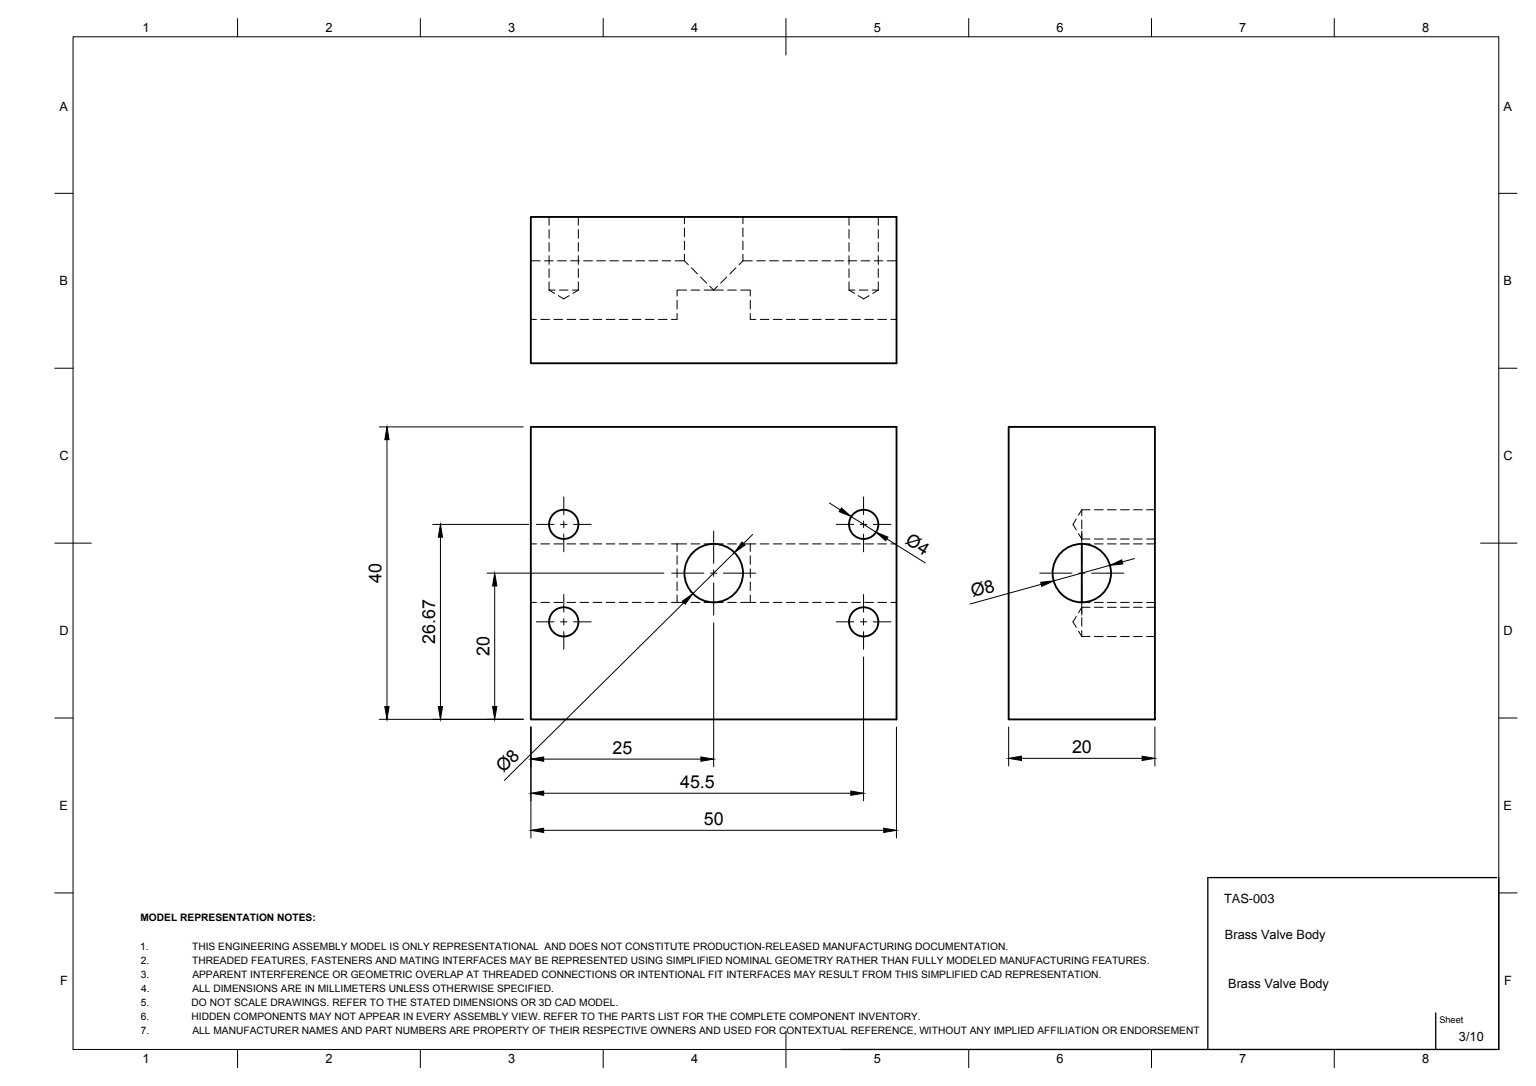
ISO-10303-21;
HEADER;
/* Generated by software containing ST-Developer
 * from STEP Tools, Inc. (www.steptools.com) 
 */

FILE_DESCRIPTION(
/* description */ ('STEP AP214'),
/* implementation_level */ '2;1');

FILE_NAME(
/* name */ 'Brass Valve Body.step',
/* time_stamp */ '2026-11-04T19:43:37-08:00',
/* author */ (''),
/* organization */ (''),
/* preprocessor_version */ 'ST-DEVELOPER v20.2',
/* originating_system */ 'Autodesk Translation Framework v15.17.0.0',
/* authorisation */ '');

FILE_SCHEMA (('AUTOMOTIVE_DESIGN { 1 0 10303 214 3 1 1 }'));
ENDSEC;

DATA;
#10=MECHANICAL_DESIGN_GEOMETRIC_PRESENTATION_REPRESENTATION('',(#115),#7627);
#97=SHAPE_REPRESENTATION_RELATIONSHIP('SRR','None',#7665,#106);
#106=ADVANCED_BREP_SHAPE_REPRESENTATION('',(#136),#7618);
#115=STYLED_ITEM('',(#7719),#136);
#136=MANIFOLD_SOLID_BREP('Body1',#2413);
#157=FACE_BOUND('',#474,.T.);
#158=FACE_BOUND('',#476,.T.);
#159=FACE_BOUND('',#479,.T.);
#160=FACE_BOUND('',#480,.T.);
#161=FACE_BOUND('',#481,.T.);
#162=FACE_BOUND('',#482,.T.);
#163=FACE_BOUND('',#483,.T.);
#191=PLANE('',#2563);
#192=PLANE('',#2564);
#193=PLANE('',#2565);
#194=PLANE('',#2566);
#195=PLANE('',#2567);
#196=PLANE('',#2568);
#197=PLANE('',#2569);
#198=PLANE('',#2570);
#199=PLANE('',#2571);
#252=ELLIPSE('',#2553,5.6568542494923,3.99999999999995);
#253=ELLIPSE('',#2554,5.65685424949242,4.00000000000003);
#254=ELLIPSE('',#2556,5.65685424949242,4.00000000000003);
#255=CYLINDRICAL_SURFACE('',#2538,2.);
#256=CYLINDRICAL_SURFACE('',#2542,2.);
#257=CYLINDRICAL_SURFACE('',#2546,2.);
#258=CYLINDRICAL_SURFACE('',#2550,2.);
#259=CYLINDRICAL_SURFACE('',#2552,4.);
#260=CYLINDRICAL_SURFACE('',#2557,4.);
#261=CYLINDRICAL_SURFACE('',#2560,4.);
#308=FACE_OUTER_BOUND('',#462,.T.);
#309=FACE_OUTER_BOUND('',#463,.T.);
#310=FACE_OUTER_BOUND('',#464,.T.);
#311=FACE_OUTER_BOUND('',#465,.T.);
#312=FACE_OUTER_BOUND('',#466,.T.);
#313=FACE_OUTER_BOUND('',#467,.T.);
#314=FACE_OUTER_BOUND('',#468,.T.);
#315=FACE_OUTER_BOUND('',#469,.T.);
#316=FACE_OUTER_BOUND('',#470,.T.);
#317=FACE_OUTER_BOUND('',#471,.T.);
#318=FACE_OUTER_BOUND('',#472,.T.);
#319=FACE_OUTER_BOUND('',#473,.T.);
#320=FACE_OUTER_BOUND('',#475,.T.);
#321=FACE_OUTER_BOUND('',#477,.T.);
#322=FACE_OUTER_BOUND('',#478,.T.);
#323=FACE_OUTER_BOUND('',#484,.T.);
#324=FACE_OUTER_BOUND('',#485,.T.);
#325=FACE_OUTER_BOUND('',#486,.T.);
#326=FACE_OUTER_BOUND('',#487,.T.);
#327=FACE_OUTER_BOUND('',#488,.T.);
#462=EDGE_LOOP('',(#1621,#1622,#1623));
#463=EDGE_LOOP('',(#1624,#1625,#1626,#1627));
#464=EDGE_LOOP('',(#1628,#1629,#1630));
#465=EDGE_LOOP('',(#1631,#1632,#1633,#1634));
#466=EDGE_LOOP('',(#1635,#1636,#1637));
#467=EDGE_LOOP('',(#1638,#1639,#1640,#1641));
#468=EDGE_LOOP('',(#1642,#1643,#1644));
#469=EDGE_LOOP('',(#1645,#1646,#1647,#1648));
#470=EDGE_LOOP('',(#1649,#1650,#1651,#1652,#1653,#1654));
#471=EDGE_LOOP('',(#1655,#1656,#1657,#1658,#1659,#1660,#1661,#1662));
#472=EDGE_LOOP('',(#1663,#1664,#1665,#1666,#1667,#1668,#1669));
#473=EDGE_LOOP('',(#1670,#1671,#1672,#1673));
#474=EDGE_LOOP('',(#1674));
#475=EDGE_LOOP('',(#1675,#1676,#1677,#1678));
#476=EDGE_LOOP('',(#1679));
#477=EDGE_LOOP('',(#1680,#1681,#1682,#1683));
#478=EDGE_LOOP('',(#1684,#1685,#1686,#1687));
#479=EDGE_LOOP('',(#1688));
#480=EDGE_LOOP('',(#1689));
#481=EDGE_LOOP('',(#1690));
#482=EDGE_LOOP('',(#1691));
#483=EDGE_LOOP('',(#1692));
#484=EDGE_LOOP('',(#1693,#1694,#1695,#1696));
#485=EDGE_LOOP('',(#1697,#1698,#1699,#1700));
#486=EDGE_LOOP('',(#1701,#1702));
#487=EDGE_LOOP('',(#1703,#1704));
#488=EDGE_LOOP('',(#1705,#1706,#1707,#1708,#1709,#1710));
#650=CIRCLE('',#2537,2.);
#651=CIRCLE('',#2539,2.);
#652=CIRCLE('',#2541,2.);
#653=CIRCLE('',#2543,2.);
#654=CIRCLE('',#2545,2.);
#655=CIRCLE('',#2547,2.);
#656=CIRCLE('',#2549,2.);
#657=CIRCLE('',#2551,2.);
#658=CIRCLE('',#2555,4.);
#659=CIRCLE('',#2558,4.);
#660=CIRCLE('',#2559,4.);
#661=CIRCLE('',#2561,4.);
#662=CIRCLE('',#2562,4.);
#803=LINE('',#3685,#959);
#804=LINE('',#3689,#960);
#805=LINE('',#3694,#961);
#806=LINE('',#3698,#962);
#807=LINE('',#3703,#963);
#808=LINE('',#3707,#964);
#809=LINE('',#3712,#965);
#810=LINE('',#3716,#966);
#811=LINE('',#3725,#967);
#812=LINE('',#3733,#968);
#813=LINE('',#3735,#969);
#814=LINE('',#3736,#970);
#815=LINE('',#3741,#971);
#816=LINE('',#3744,#972);
#817=LINE('',#3745,#973);
#818=LINE('',#3749,#974);
#819=LINE('',#3751,#975);
#820=LINE('',#3753,#976);
#821=LINE('',#3754,#977);
#822=LINE('',#3758,#978);
#823=LINE('',#3760,#979);
#824=LINE('',#3762,#980);
#825=LINE('',#3763,#981);
#826=LINE('',#3765,#982);
#827=LINE('',#3766,#983);
#828=LINE('',#3768,#984);
#829=LINE('',#3770,#985);
#830=LINE('',#3773,#986);
#831=LINE('',#3775,#987);
#959=VECTOR('',#2870,2.);
#960=VECTOR('',#2875,2.);
#961=VECTOR('',#2880,2.);
#962=VECTOR('',#2885,2.);
#963=VECTOR('',#2890,2.);
#964=VECTOR('',#2895,2.);
#965=VECTOR('',#2900,2.);
#966=VECTOR('',#2905,2.);
#967=VECTOR('',#2914,4.);
#968=VECTOR('',#2923,4.);
#969=VECTOR('',#2926,1000.);
#970=VECTOR('',#2927,1000.);
#971=VECTOR('',#2932,4.);
#972=VECTOR('',#2935,1000.);
#973=VECTOR('',#2936,1000.);
#974=VECTOR('',#2939,1000.);
#975=VECTOR('',#2940,1000.);
#976=VECTOR('',#2941,1000.);
#977=VECTOR('',#2942,1000.);
#978=VECTOR('',#2945,1000.);
#979=VECTOR('',#2946,1000.);
#980=VECTOR('',#2947,1000.);
#981=VECTOR('',#2948,1000.);
#982=VECTOR('',#2951,1000.);
#983=VECTOR('',#2952,1000.);
#984=VECTOR('',#2955,1000.);
#985=VECTOR('',#2958,1000.);
#986=VECTOR('',#2963,1000.);
#987=VECTOR('',#2966,1000.);
#1115=VERTEX_POINT('',#3683);
#1116=VERTEX_POINT('',#3684);
#1117=VERTEX_POINT('',#3688);
#1118=VERTEX_POINT('',#3692);
#1119=VERTEX_POINT('',#3693);
#1120=VERTEX_POINT('',#3697);
#1121=VERTEX_POINT('',#3701);
#1122=VERTEX_POINT('',#3702);
#1123=VERTEX_POINT('',#3706);
#1124=VERTEX_POINT('',#3710);
#1125=VERTEX_POINT('',#3711);
#1126=VERTEX_POINT('',#3715);
#1127=VERTEX_POINT('',#3719);
#1128=VERTEX_POINT('',#3720);
#1129=VERTEX_POINT('',#3722);
#1130=VERTEX_POINT('',#3724);
#1131=VERTEX_POINT('',#3729);
#1132=VERTEX_POINT('',#3730);
#1133=VERTEX_POINT('',#3732);
#1134=VERTEX_POINT('',#3738);
#1135=VERTEX_POINT('',#3740);
#1136=VERTEX_POINT('',#3742);
#1137=VERTEX_POINT('',#3747);
#1138=VERTEX_POINT('',#3748);
#1139=VERTEX_POINT('',#3750);
#1140=VERTEX_POINT('',#3752);
#1141=VERTEX_POINT('',#3756);
#1142=VERTEX_POINT('',#3757);
#1143=VERTEX_POINT('',#3759);
#1144=VERTEX_POINT('',#3761);
#1305=EDGE_CURVE('',#1115,#1116,#803,.T.);
#1306=EDGE_CURVE('',#1116,#1116,#650,.T.);
#1307=EDGE_CURVE('',#1116,#1117,#804,.T.);
#1308=EDGE_CURVE('',#1117,#1117,#651,.T.);
#1309=EDGE_CURVE('',#1118,#1119,#805,.T.);
#1310=EDGE_CURVE('',#1119,#1119,#652,.T.);
#1311=EDGE_CURVE('',#1119,#1120,#806,.T.);
#1312=EDGE_CURVE('',#1120,#1120,#653,.T.);
#1313=EDGE_CURVE('',#1121,#1122,#807,.T.);
#1314=EDGE_CURVE('',#1122,#1122,#654,.T.);
#1315=EDGE_CURVE('',#1122,#1123,#808,.T.);
#1316=EDGE_CURVE('',#1123,#1123,#655,.T.);
#1317=EDGE_CURVE('',#1124,#1125,#809,.T.);
#1318=EDGE_CURVE('',#1125,#1125,#656,.T.);
#1319=EDGE_CURVE('',#1125,#1126,#810,.T.);
#1320=EDGE_CURVE('',#1126,#1126,#657,.T.);
#1321=EDGE_CURVE('',#1127,#1128,#252,.T.);
#1322=EDGE_CURVE('',#1129,#1127,#253,.T.);
#1323=EDGE_CURVE('',#1129,#1130,#811,.T.);
#1324=EDGE_CURVE('',#1130,#1130,#658,.T.);
#1325=EDGE_CURVE('',#1128,#1129,#254,.T.);
#1326=EDGE_CURVE('',#1131,#1132,#659,.T.);
#1327=EDGE_CURVE('',#1131,#1133,#812,.T.);
#1328=EDGE_CURVE('',#1133,#1133,#660,.T.);
#1329=EDGE_CURVE('',#1128,#1131,#813,.T.);
#1330=EDGE_CURVE('',#1132,#1127,#814,.T.);
#1331=EDGE_CURVE('',#1134,#1134,#661,.T.);
#1332=EDGE_CURVE('',#1134,#1135,#815,.T.);
#1333=EDGE_CURVE('',#1136,#1135,#662,.T.);
#1334=EDGE_CURVE('',#1127,#1136,#816,.T.);
#1335=EDGE_CURVE('',#1135,#1128,#817,.T.);
#1336=EDGE_CURVE('',#1137,#1138,#818,.T.);
#1337=EDGE_CURVE('',#1138,#1139,#819,.T.);
#1338=EDGE_CURVE('',#1139,#1140,#820,.T.);
#1339=EDGE_CURVE('',#1140,#1137,#821,.T.);
#1340=EDGE_CURVE('',#1141,#1142,#822,.T.);
#1341=EDGE_CURVE('',#1143,#1141,#823,.T.);
#1342=EDGE_CURVE('',#1144,#1143,#824,.T.);
#1343=EDGE_CURVE('',#1142,#1144,#825,.T.);
#1344=EDGE_CURVE('',#1138,#1142,#826,.T.);
#1345=EDGE_CURVE('',#1137,#1141,#827,.T.);
#1346=EDGE_CURVE('',#1139,#1144,#828,.T.);
#1347=EDGE_CURVE('',#1140,#1143,#829,.T.);
#1348=EDGE_CURVE('',#1132,#1131,#830,.T.);
#1349=EDGE_CURVE('',#1135,#1136,#831,.T.);
#1621=ORIENTED_EDGE('',*,*,#1305,.T.);
#1622=ORIENTED_EDGE('',*,*,#1306,.T.);
#1623=ORIENTED_EDGE('',*,*,#1305,.F.);
#1624=ORIENTED_EDGE('',*,*,#1306,.F.);
#1625=ORIENTED_EDGE('',*,*,#1307,.T.);
#1626=ORIENTED_EDGE('',*,*,#1308,.T.);
#1627=ORIENTED_EDGE('',*,*,#1307,.F.);
#1628=ORIENTED_EDGE('',*,*,#1309,.T.);
#1629=ORIENTED_EDGE('',*,*,#1310,.T.);
#1630=ORIENTED_EDGE('',*,*,#1309,.F.);
#1631=ORIENTED_EDGE('',*,*,#1310,.F.);
#1632=ORIENTED_EDGE('',*,*,#1311,.T.);
#1633=ORIENTED_EDGE('',*,*,#1312,.T.);
#1634=ORIENTED_EDGE('',*,*,#1311,.F.);
#1635=ORIENTED_EDGE('',*,*,#1313,.T.);
#1636=ORIENTED_EDGE('',*,*,#1314,.T.);
#1637=ORIENTED_EDGE('',*,*,#1313,.F.);
#1638=ORIENTED_EDGE('',*,*,#1314,.F.);
#1639=ORIENTED_EDGE('',*,*,#1315,.T.);
#1640=ORIENTED_EDGE('',*,*,#1316,.T.);
#1641=ORIENTED_EDGE('',*,*,#1315,.F.);
#1642=ORIENTED_EDGE('',*,*,#1317,.T.);
#1643=ORIENTED_EDGE('',*,*,#1318,.T.);
#1644=ORIENTED_EDGE('',*,*,#1317,.F.);
#1645=ORIENTED_EDGE('',*,*,#1318,.F.);
#1646=ORIENTED_EDGE('',*,*,#1319,.T.);
#1647=ORIENTED_EDGE('',*,*,#1320,.T.);
#1648=ORIENTED_EDGE('',*,*,#1319,.F.);
#1649=ORIENTED_EDGE('',*,*,#1321,.F.);
#1650=ORIENTED_EDGE('',*,*,#1322,.F.);
#1651=ORIENTED_EDGE('',*,*,#1323,.T.);
#1652=ORIENTED_EDGE('',*,*,#1324,.T.);
#1653=ORIENTED_EDGE('',*,*,#1323,.F.);
#1654=ORIENTED_EDGE('',*,*,#1325,.F.);
#1655=ORIENTED_EDGE('',*,*,#1326,.F.);
#1656=ORIENTED_EDGE('',*,*,#1327,.T.);
#1657=ORIENTED_EDGE('',*,*,#1328,.F.);
#1658=ORIENTED_EDGE('',*,*,#1327,.F.);
#1659=ORIENTED_EDGE('',*,*,#1329,.F.);
#1660=ORIENTED_EDGE('',*,*,#1325,.T.);
#1661=ORIENTED_EDGE('',*,*,#1322,.T.);
#1662=ORIENTED_EDGE('',*,*,#1330,.F.);
#1663=ORIENTED_EDGE('',*,*,#1331,.T.);
#1664=ORIENTED_EDGE('',*,*,#1332,.T.);
#1665=ORIENTED_EDGE('',*,*,#1333,.F.);
#1666=ORIENTED_EDGE('',*,*,#1334,.F.);
#1667=ORIENTED_EDGE('',*,*,#1321,.T.);
#1668=ORIENTED_EDGE('',*,*,#1335,.F.);
#1669=ORIENTED_EDGE('',*,*,#1332,.F.);
#1670=ORIENTED_EDGE('',*,*,#1336,.T.);
#1671=ORIENTED_EDGE('',*,*,#1337,.T.);
#1672=ORIENTED_EDGE('',*,*,#1338,.T.);
#1673=ORIENTED_EDGE('',*,*,#1339,.T.);
#1674=ORIENTED_EDGE('',*,*,#1331,.F.);
#1675=ORIENTED_EDGE('',*,*,#1340,.F.);
#1676=ORIENTED_EDGE('',*,*,#1341,.F.);
#1677=ORIENTED_EDGE('',*,*,#1342,.F.);
#1678=ORIENTED_EDGE('',*,*,#1343,.F.);
#1679=ORIENTED_EDGE('',*,*,#1328,.T.);
#1680=ORIENTED_EDGE('',*,*,#1340,.T.);
#1681=ORIENTED_EDGE('',*,*,#1344,.F.);
#1682=ORIENTED_EDGE('',*,*,#1336,.F.);
#1683=ORIENTED_EDGE('',*,*,#1345,.T.);
#1684=ORIENTED_EDGE('',*,*,#1343,.T.);
#1685=ORIENTED_EDGE('',*,*,#1346,.F.);
#1686=ORIENTED_EDGE('',*,*,#1337,.F.);
#1687=ORIENTED_EDGE('',*,*,#1344,.T.);
#1688=ORIENTED_EDGE('',*,*,#1308,.F.);
#1689=ORIENTED_EDGE('',*,*,#1312,.F.);
#1690=ORIENTED_EDGE('',*,*,#1316,.F.);
#1691=ORIENTED_EDGE('',*,*,#1320,.F.);
#1692=ORIENTED_EDGE('',*,*,#1324,.F.);
#1693=ORIENTED_EDGE('',*,*,#1342,.T.);
#1694=ORIENTED_EDGE('',*,*,#1347,.F.);
#1695=ORIENTED_EDGE('',*,*,#1338,.F.);
#1696=ORIENTED_EDGE('',*,*,#1346,.T.);
#1697=ORIENTED_EDGE('',*,*,#1341,.T.);
#1698=ORIENTED_EDGE('',*,*,#1345,.F.);
#1699=ORIENTED_EDGE('',*,*,#1339,.F.);
#1700=ORIENTED_EDGE('',*,*,#1347,.T.);
#1701=ORIENTED_EDGE('',*,*,#1348,.T.);
#1702=ORIENTED_EDGE('',*,*,#1326,.T.);
#1703=ORIENTED_EDGE('',*,*,#1349,.T.);
#1704=ORIENTED_EDGE('',*,*,#1333,.T.);
#1705=ORIENTED_EDGE('',*,*,#1349,.F.);
#1706=ORIENTED_EDGE('',*,*,#1335,.T.);
#1707=ORIENTED_EDGE('',*,*,#1329,.T.);
#1708=ORIENTED_EDGE('',*,*,#1348,.F.);
#1709=ORIENTED_EDGE('',*,*,#1330,.T.);
#1710=ORIENTED_EDGE('',*,*,#1334,.T.);
#2253=CONICAL_SURFACE('',#2536,2.,1.02974426);
#2254=CONICAL_SURFACE('',#2540,2.,1.02974426);
#2255=CONICAL_SURFACE('',#2544,2.,1.02974426);
#2256=CONICAL_SURFACE('',#2548,2.,1.02974426);
#2259=ADVANCED_FACE('',(#308),#2253,.F.);
#2260=ADVANCED_FACE('',(#309),#255,.F.);
#2261=ADVANCED_FACE('',(#310),#2254,.F.);
#2262=ADVANCED_FACE('',(#311),#256,.F.);
#2263=ADVANCED_FACE('',(#312),#2255,.F.);
#2264=ADVANCED_FACE('',(#313),#257,.F.);
#2265=ADVANCED_FACE('',(#314),#2256,.F.);
#2266=ADVANCED_FACE('',(#315),#258,.F.);
#2267=ADVANCED_FACE('',(#316),#259,.F.);
#2268=ADVANCED_FACE('',(#317),#260,.F.);
#2269=ADVANCED_FACE('',(#318),#261,.F.);
#2270=ADVANCED_FACE('',(#319,#157),#191,.F.);
#2271=ADVANCED_FACE('',(#320,#158),#192,.T.);
#2272=ADVANCED_FACE('',(#321),#193,.F.);
#2273=ADVANCED_FACE('',(#322,#159,#160,#161,#162,#163),#194,.F.);
#2274=ADVANCED_FACE('',(#323),#195,.F.);
#2275=ADVANCED_FACE('',(#324),#196,.F.);
#2276=ADVANCED_FACE('',(#325),#197,.T.);
#2277=ADVANCED_FACE('',(#326),#198,.T.);
#2278=ADVANCED_FACE('',(#327),#199,.T.);
#2413=CLOSED_SHELL('',(#2259,#2260,#2261,#2262,#2263,#2264,#2265,#2266,
#2267,#2268,#2269,#2270,#2271,#2272,#2273,#2274,#2275,#2276,#2277,#2278));
#2535=AXIS2_PLACEMENT_3D('',#3681,#2866,#2867);
#2536=AXIS2_PLACEMENT_3D('',#3682,#2868,#2869);
#2537=AXIS2_PLACEMENT_3D('',#3686,#2871,#2872);
#2538=AXIS2_PLACEMENT_3D('',#3687,#2873,#2874);
#2539=AXIS2_PLACEMENT_3D('',#3690,#2876,#2877);
#2540=AXIS2_PLACEMENT_3D('',#3691,#2878,#2879);
#2541=AXIS2_PLACEMENT_3D('',#3695,#2881,#2882);
#2542=AXIS2_PLACEMENT_3D('',#3696,#2883,#2884);
#2543=AXIS2_PLACEMENT_3D('',#3699,#2886,#2887);
#2544=AXIS2_PLACEMENT_3D('',#3700,#2888,#2889);
#2545=AXIS2_PLACEMENT_3D('',#3704,#2891,#2892);
#2546=AXIS2_PLACEMENT_3D('',#3705,#2893,#2894);
#2547=AXIS2_PLACEMENT_3D('',#3708,#2896,#2897);
#2548=AXIS2_PLACEMENT_3D('',#3709,#2898,#2899);
#2549=AXIS2_PLACEMENT_3D('',#3713,#2901,#2902);
#2550=AXIS2_PLACEMENT_3D('',#3714,#2903,#2904);
#2551=AXIS2_PLACEMENT_3D('',#3717,#2906,#2907);
#2552=AXIS2_PLACEMENT_3D('',#3718,#2908,#2909);
#2553=AXIS2_PLACEMENT_3D('',#3721,#2910,#2911);
#2554=AXIS2_PLACEMENT_3D('',#3723,#2912,#2913);
#2555=AXIS2_PLACEMENT_3D('',#3726,#2915,#2916);
#2556=AXIS2_PLACEMENT_3D('',#3727,#2917,#2918);
#2557=AXIS2_PLACEMENT_3D('',#3728,#2919,#2920);
#2558=AXIS2_PLACEMENT_3D('',#3731,#2921,#2922);
#2559=AXIS2_PLACEMENT_3D('',#3734,#2924,#2925);
#2560=AXIS2_PLACEMENT_3D('',#3737,#2928,#2929);
#2561=AXIS2_PLACEMENT_3D('',#3739,#2930,#2931);
#2562=AXIS2_PLACEMENT_3D('',#3743,#2933,#2934);
#2563=AXIS2_PLACEMENT_3D('',#3746,#2937,#2938);
#2564=AXIS2_PLACEMENT_3D('',#3755,#2943,#2944);
#2565=AXIS2_PLACEMENT_3D('',#3764,#2949,#2950);
#2566=AXIS2_PLACEMENT_3D('',#3767,#2953,#2954);
#2567=AXIS2_PLACEMENT_3D('',#3769,#2956,#2957);
#2568=AXIS2_PLACEMENT_3D('',#3771,#2959,#2960);
#2569=AXIS2_PLACEMENT_3D('',#3772,#2961,#2962);
#2570=AXIS2_PLACEMENT_3D('',#3774,#2964,#2965);
#2571=AXIS2_PLACEMENT_3D('',#3776,#2967,#2968);
#2866=DIRECTION('axis',(0.,0.,1.));
#2867=DIRECTION('refdir',(1.,0.,0.));
#2868=DIRECTION('center_axis',(0.,1.,0.));
#2869=DIRECTION('ref_axis',(0.,0.,1.));
#2870=DIRECTION('',(-1.04972719197331E-16,0.515038073775726,-0.857167301383686));
#2871=DIRECTION('center_axis',(0.,1.,0.));
#2872=DIRECTION('ref_axis',(0.,0.,1.));
#2873=DIRECTION('center_axis',(0.,1.,0.));
#2874=DIRECTION('ref_axis',(0.,0.,1.));
#2875=DIRECTION('',(0.,1.,0.));
#2876=DIRECTION('center_axis',(0.,1.,0.));
#2877=DIRECTION('ref_axis',(0.,0.,1.));
#2878=DIRECTION('center_axis',(0.,1.,0.));
#2879=DIRECTION('ref_axis',(0.,0.,1.));
#2880=DIRECTION('',(-1.04972719197331E-16,0.515038073775726,-0.857167301383686));
#2881=DIRECTION('center_axis',(0.,1.,0.));
#2882=DIRECTION('ref_axis',(0.,0.,1.));
#2883=DIRECTION('center_axis',(0.,1.,0.));
#2884=DIRECTION('ref_axis',(0.,0.,1.));
#2885=DIRECTION('',(0.,1.,0.));
#2886=DIRECTION('center_axis',(0.,1.,0.));
#2887=DIRECTION('ref_axis',(0.,0.,1.));
#2888=DIRECTION('center_axis',(0.,1.,0.));
#2889=DIRECTION('ref_axis',(0.,0.,1.));
#2890=DIRECTION('',(-1.04972719197331E-16,0.515038073775726,-0.857167301383686));
#2891=DIRECTION('center_axis',(0.,1.,0.));
#2892=DIRECTION('ref_axis',(0.,0.,1.));
#2893=DIRECTION('center_axis',(0.,1.,0.));
#2894=DIRECTION('ref_axis',(0.,0.,1.));
#2895=DIRECTION('',(0.,1.,0.));
#2896=DIRECTION('center_axis',(0.,1.,0.));
#2897=DIRECTION('ref_axis',(0.,0.,1.));
#2898=DIRECTION('center_axis',(0.,1.,0.));
#2899=DIRECTION('ref_axis',(0.,0.,1.));
#2900=DIRECTION('',(-1.04972719197331E-16,0.515038073775726,-0.857167301383686));
#2901=DIRECTION('center_axis',(0.,1.,0.));
#2902=DIRECTION('ref_axis',(0.,0.,1.));
#2903=DIRECTION('center_axis',(0.,1.,0.));
#2904=DIRECTION('ref_axis',(0.,0.,1.));
#2905=DIRECTION('',(0.,1.,0.));
#2906=DIRECTION('center_axis',(0.,1.,0.));
#2907=DIRECTION('ref_axis',(0.,0.,1.));
#2908=DIRECTION('center_axis',(0.,1.,0.));
#2909=DIRECTION('ref_axis',(0.,0.,1.));
#2910=DIRECTION('center_axis',(0.,0.707106781186548,-0.707106781186548));
#2911=DIRECTION('ref_axis',(1.76988781740397E-14,0.707106781186548,0.707106781186548));
#2912=DIRECTION('center_axis',(0.,0.707106781186548,0.707106781186548));
#2913=DIRECTION('ref_axis',(7.96449517831793E-15,-0.707106781186548,0.707106781186548));
#2914=DIRECTION('',(0.,1.,0.));
#2915=DIRECTION('center_axis',(0.,1.,0.));
#2916=DIRECTION('ref_axis',(0.,0.,1.));
#2917=DIRECTION('center_axis',(0.,0.707106781186548,0.707106781186548));
#2918=DIRECTION('ref_axis',(7.96449517831793E-15,-0.707106781186548,0.707106781186548));
#2919=DIRECTION('center_axis',(0.,0.,-1.));
#2920=DIRECTION('ref_axis',(-1.,0.,0.));
#2921=DIRECTION('center_axis',(0.,0.,-1.));
#2922=DIRECTION('ref_axis',(-1.,0.,0.));
#2923=DIRECTION('',(0.,0.,-1.));
#2924=DIRECTION('center_axis',(0.,0.,1.));
#2925=DIRECTION('ref_axis',(1.,0.,0.));
#2926=DIRECTION('',(0.,0.,-1.));
#2927=DIRECTION('',(0.,0.,1.));
#2928=DIRECTION('center_axis',(0.,0.,-1.));
#2929=DIRECTION('ref_axis',(-1.,0.,0.));
#2930=DIRECTION('center_axis',(0.,0.,1.));
#2931=DIRECTION('ref_axis',(1.,0.,0.));
#2932=DIRECTION('',(0.,0.,-1.));
#2933=DIRECTION('center_axis',(8.67361737988403E-17,0.,1.));
#2934=DIRECTION('ref_axis',(1.,0.,-8.67361737988404E-17));
#2935=DIRECTION('',(0.,0.,1.));
#2936=DIRECTION('',(0.,0.,-1.));
#2937=DIRECTION('center_axis',(0.,0.,-1.));
#2938=DIRECTION('ref_axis',(-1.,0.,0.));
#2939=DIRECTION('',(0.,1.,0.));
#2940=DIRECTION('',(-1.,0.,0.));
#2941=DIRECTION('',(0.,-1.,0.));
#2942=DIRECTION('',(1.,0.,0.));
#2943=DIRECTION('center_axis',(0.,0.,-1.));
#2944=DIRECTION('ref_axis',(-1.,0.,0.));
#2945=DIRECTION('',(0.,1.,0.));
#2946=DIRECTION('',(1.,0.,0.));
#2947=DIRECTION('',(0.,-1.,0.));
#2948=DIRECTION('',(-1.,0.,0.));
#2949=DIRECTION('center_axis',(-1.,0.,0.));
#2950=DIRECTION('ref_axis',(0.,0.,1.));
#2951=DIRECTION('',(0.,0.,-1.));
#2952=DIRECTION('',(0.,0.,-1.));
#2953=DIRECTION('center_axis',(0.,-1.,0.));
#2954=DIRECTION('ref_axis',(0.,0.,-1.));
#2955=DIRECTION('',(0.,0.,-1.));
#2956=DIRECTION('center_axis',(1.,0.,0.));
#2957=DIRECTION('ref_axis',(0.,0.,-1.));
#2958=DIRECTION('',(0.,0.,-1.));
#2959=DIRECTION('center_axis',(0.,1.,0.));
#2960=DIRECTION('ref_axis',(0.,0.,1.));
#2961=DIRECTION('center_axis',(0.,0.,-1.));
#2962=DIRECTION('ref_axis',(-1.,0.,0.));
#2963=DIRECTION('',(1.,0.,0.));
#2964=DIRECTION('center_axis',(8.67361737988403E-17,0.,1.));
#2965=DIRECTION('ref_axis',(1.,0.,-8.67361737988404E-17));
#2966=DIRECTION('',(-1.,0.,8.67361737988404E-17));
#2967=DIRECTION('center_axis',(0.,1.,0.));
#2968=DIRECTION('ref_axis',(0.,0.,1.));
#3681=CARTESIAN_POINT('',(0.,0.,0.));
#3682=CARTESIAN_POINT('Origin',(-6.66666666666667,0.,20.5));
#3683=CARTESIAN_POINT('',(-6.66666666666667,-1.20172123445289,20.5));
#3684=CARTESIAN_POINT('',(-6.66666666666667,0.,18.5));
#3685=CARTESIAN_POINT('',(-6.66666666666667,0.,18.5));
#3686=CARTESIAN_POINT('Origin',(-6.66666666666667,0.,20.5));
#3687=CARTESIAN_POINT('Origin',(-6.66666666666667,10.,20.5));
#3688=CARTESIAN_POINT('',(-6.66666666666667,10.,18.5));
#3689=CARTESIAN_POINT('',(-6.66666666666667,10.,18.5));
#3690=CARTESIAN_POINT('Origin',(-6.66666666666667,10.,20.5));
#3691=CARTESIAN_POINT('Origin',(6.66666666666666,0.,20.5));
#3692=CARTESIAN_POINT('',(6.66666666666666,-1.20172123445289,20.5));
#3693=CARTESIAN_POINT('',(6.66666666666666,0.,18.5));
#3694=CARTESIAN_POINT('',(6.66666666666666,0.,18.5));
#3695=CARTESIAN_POINT('Origin',(6.66666666666666,0.,20.5));
#3696=CARTESIAN_POINT('Origin',(6.66666666666666,10.,20.5));
#3697=CARTESIAN_POINT('',(6.66666666666666,10.,18.5));
#3698=CARTESIAN_POINT('',(6.66666666666666,10.,18.5));
#3699=CARTESIAN_POINT('Origin',(6.66666666666666,10.,20.5));
#3700=CARTESIAN_POINT('Origin',(6.66666666666666,0.,-20.5));
#3701=CARTESIAN_POINT('',(6.66666666666666,-1.20172123445289,-20.5));
#3702=CARTESIAN_POINT('',(6.66666666666666,0.,-22.5));
#3703=CARTESIAN_POINT('',(6.66666666666666,0.,-22.5));
#3704=CARTESIAN_POINT('Origin',(6.66666666666666,0.,-20.5));
#3705=CARTESIAN_POINT('Origin',(6.66666666666666,10.,-20.5));
#3706=CARTESIAN_POINT('',(6.66666666666666,10.,-22.5));
#3707=CARTESIAN_POINT('',(6.66666666666666,10.,-22.5));
#3708=CARTESIAN_POINT('Origin',(6.66666666666666,10.,-20.5));
#3709=CARTESIAN_POINT('Origin',(-6.66666666666667,0.,-20.5));
#3710=CARTESIAN_POINT('',(-6.66666666666667,-1.20172123445289,-20.5));
#3711=CARTESIAN_POINT('',(-6.66666666666667,0.,-22.5));
#3712=CARTESIAN_POINT('',(-6.66666666666667,0.,-22.5));
#3713=CARTESIAN_POINT('Origin',(-6.66666666666667,0.,-20.5));
#3714=CARTESIAN_POINT('Origin',(-6.66666666666667,10.,-20.5));
#3715=CARTESIAN_POINT('',(-6.66666666666667,10.,-22.5));
#3716=CARTESIAN_POINT('',(-6.66666666666667,10.,-22.5));
#3717=CARTESIAN_POINT('Origin',(-6.66666666666667,10.,-20.5));
#3718=CARTESIAN_POINT('Origin',(0.,-10.001,0.));
#3719=CARTESIAN_POINT('',(-4.,6.93889390390723E-15,0.));
#3720=CARTESIAN_POINT('',(4.,6.93889390390723E-15,0.));
#3721=CARTESIAN_POINT('Origin',(-5.44009282066327E-14,6.53255536936271E-14,
5.83866597897199E-14));
#3722=CARTESIAN_POINT('',(-4.8985871965897E-16,4.00000000000001,-4.));
#3723=CARTESIAN_POINT('Origin',(2.8461243742395E-14,-1.94289029309402E-14,
2.66453525910038E-14));
#3724=CARTESIAN_POINT('',(-4.89858719658941E-16,10.,-4.));
#3725=CARTESIAN_POINT('',(-4.89858719658941E-16,-10.001,-4.));
#3726=CARTESIAN_POINT('Origin',(0.,10.,0.));
#3727=CARTESIAN_POINT('Origin',(2.8461243742395E-14,-1.94289029309402E-14,
2.66453525910038E-14));
#3728=CARTESIAN_POINT('Origin',(-6.93889390390723E-15,6.93889390390723E-15,
25.));
#3729=CARTESIAN_POINT('',(3.99999999999999,0.,-5.));
#3730=CARTESIAN_POINT('',(-4.00000000000001,0.,-5.));
#3731=CARTESIAN_POINT('Origin',(-6.93889390390723E-15,6.93889390390723E-15,
-5.));
#3732=CARTESIAN_POINT('',(3.99999999999999,6.44903518424829E-15,-25.));
#3733=CARTESIAN_POINT('',(3.99999999999999,6.44903518424829E-15,25.));
#3734=CARTESIAN_POINT('Origin',(-6.93889390390723E-15,6.93889390390723E-15,
-25.));
#3735=CARTESIAN_POINT('',(3.99999999999999,0.,25.));
#3736=CARTESIAN_POINT('',(-4.00000000000001,0.,25.));
#3737=CARTESIAN_POINT('Origin',(-6.93889390390723E-15,6.93889390390723E-15,
25.));
#3738=CARTESIAN_POINT('',(3.99999999999999,6.44903518424829E-15,25.));
#3739=CARTESIAN_POINT('Origin',(-6.93889390390723E-15,6.93889390390723E-15,
25.));
#3740=CARTESIAN_POINT('',(3.99999999999999,0.,5.));
#3741=CARTESIAN_POINT('',(3.99999999999999,6.44903518424829E-15,25.));
#3742=CARTESIAN_POINT('',(-4.00000000000001,0.,5.));
#3743=CARTESIAN_POINT('Origin',(-6.93889390390723E-15,6.93889390390723E-15,
5.));
#3744=CARTESIAN_POINT('',(-4.00000000000001,0.,25.));
#3745=CARTESIAN_POINT('',(3.99999999999999,0.,25.));
#3746=CARTESIAN_POINT('Origin',(0.,0.,25.));
#3747=CARTESIAN_POINT('',(20.,-10.,25.));
#3748=CARTESIAN_POINT('',(20.,10.,25.));
#3749=CARTESIAN_POINT('',(20.,-10.,25.));
#3750=CARTESIAN_POINT('',(-20.,10.,25.));
#3751=CARTESIAN_POINT('',(-20.,10.,25.));
#3752=CARTESIAN_POINT('',(-20.,-10.,25.));
#3753=CARTESIAN_POINT('',(-20.,-10.,25.));
#3754=CARTESIAN_POINT('',(-20.,-10.,25.));
#3755=CARTESIAN_POINT('Origin',(0.,0.,-25.));
#3756=CARTESIAN_POINT('',(20.,-10.,-25.));
#3757=CARTESIAN_POINT('',(20.,10.,-25.));
#3758=CARTESIAN_POINT('',(20.,-10.,-25.));
#3759=CARTESIAN_POINT('',(-20.,-10.,-25.));
#3760=CARTESIAN_POINT('',(-20.,-10.,-25.));
#3761=CARTESIAN_POINT('',(-20.,10.,-25.));
#3762=CARTESIAN_POINT('',(-20.,-10.,-25.));
#3763=CARTESIAN_POINT('',(-20.,10.,-25.));
#3764=CARTESIAN_POINT('Origin',(20.,-10.,25.));
#3765=CARTESIAN_POINT('',(20.,10.,25.));
#3766=CARTESIAN_POINT('',(20.,-10.,25.));
#3767=CARTESIAN_POINT('Origin',(-20.,10.,25.));
#3768=CARTESIAN_POINT('',(-20.,10.,25.));
#3769=CARTESIAN_POINT('Origin',(-20.,-10.,25.));
#3770=CARTESIAN_POINT('',(-20.,-10.,25.));
#3771=CARTESIAN_POINT('Origin',(-20.,-10.,25.));
#3772=CARTESIAN_POINT('Origin',(-5.,0.,-5.));
#3773=CARTESIAN_POINT('',(-5.,0.,-5.));
#3774=CARTESIAN_POINT('Origin',(-5.,0.,5.));
#3775=CARTESIAN_POINT('',(-5.,0.,5.));
#3776=CARTESIAN_POINT('Origin',(0.,0.,0.));
#7607=UNCERTAINTY_MEASURE_WITH_UNIT(LENGTH_MEASURE(0.01),#7628,
'DISTANCE_ACCURACY_VALUE',
'Maximum model space distance between geometric entities at asserted c
onnectivities');
#7616=UNCERTAINTY_MEASURE_WITH_UNIT(LENGTH_MEASURE(0.01),#7628,
'DISTANCE_ACCURACY_VALUE',
'Maximum model space distance between geometric entities at asserted c
onnectivities');
#7618=(
GEOMETRIC_REPRESENTATION_CONTEXT(3)
GLOBAL_UNCERTAINTY_ASSIGNED_CONTEXT((#7607))
GLOBAL_UNIT_ASSIGNED_CONTEXT((#7628,#7630,#7631))
REPRESENTATION_CONTEXT('','3D')
);
#7627=(
GEOMETRIC_REPRESENTATION_CONTEXT(3)
GLOBAL_UNCERTAINTY_ASSIGNED_CONTEXT((#7616))
GLOBAL_UNIT_ASSIGNED_CONTEXT((#7628,#7630,#7631))
REPRESENTATION_CONTEXT('','3D')
);
#7628=(
LENGTH_UNIT()
NAMED_UNIT(*)
SI_UNIT(.MILLI.,.METRE.)
);
#7630=(
NAMED_UNIT(*)
PLANE_ANGLE_UNIT()
SI_UNIT($,.RADIAN.)
);
#7631=(
NAMED_UNIT(*)
SI_UNIT($,.STERADIAN.)
SOLID_ANGLE_UNIT()
);
#7633=SHAPE_DEFINITION_REPRESENTATION(#7643,#7665);
#7643=PRODUCT_DEFINITION_SHAPE('',$,#7676);
#7665=SHAPE_REPRESENTATION('',(#2535),#7618);
#7674=PRODUCT_DEFINITION_CONTEXT('part definition',#7706,'design');
#7676=PRODUCT_DEFINITION('Brass Valve Body','Brass Valve Body',#7686,#7674);
#7686=PRODUCT_DEFINITION_FORMATION('',$,#7709);
#7706=APPLICATION_CONTEXT(
'Core Data for Automotive Mechanical Design Process');
#7707=PRODUCT_CONTEXT('part definition',#7706,'mechanical');
#7709=PRODUCT('Brass Valve Body','Brass Valve Body',$,(#7707));
#7719=PRESENTATION_STYLE_ASSIGNMENT((#7725));
#7725=SURFACE_STYLE_USAGE(.BOTH.,#7731);
#7731=SURFACE_SIDE_STYLE('',(#7737));
#7737=SURFACE_STYLE_FILL_AREA(#7743);
#7743=FILL_AREA_STYLE('Opaque(20,51,87)',(#7749));
#7749=FILL_AREA_STYLE_COLOUR('Opaque(20,51,87)',#7755);
#7755=COLOUR_RGB('Opaque(20,51,87)',0.0784313725490196,0.2,0.341176470588235);
ENDSEC;
END-ISO-10303-21;
